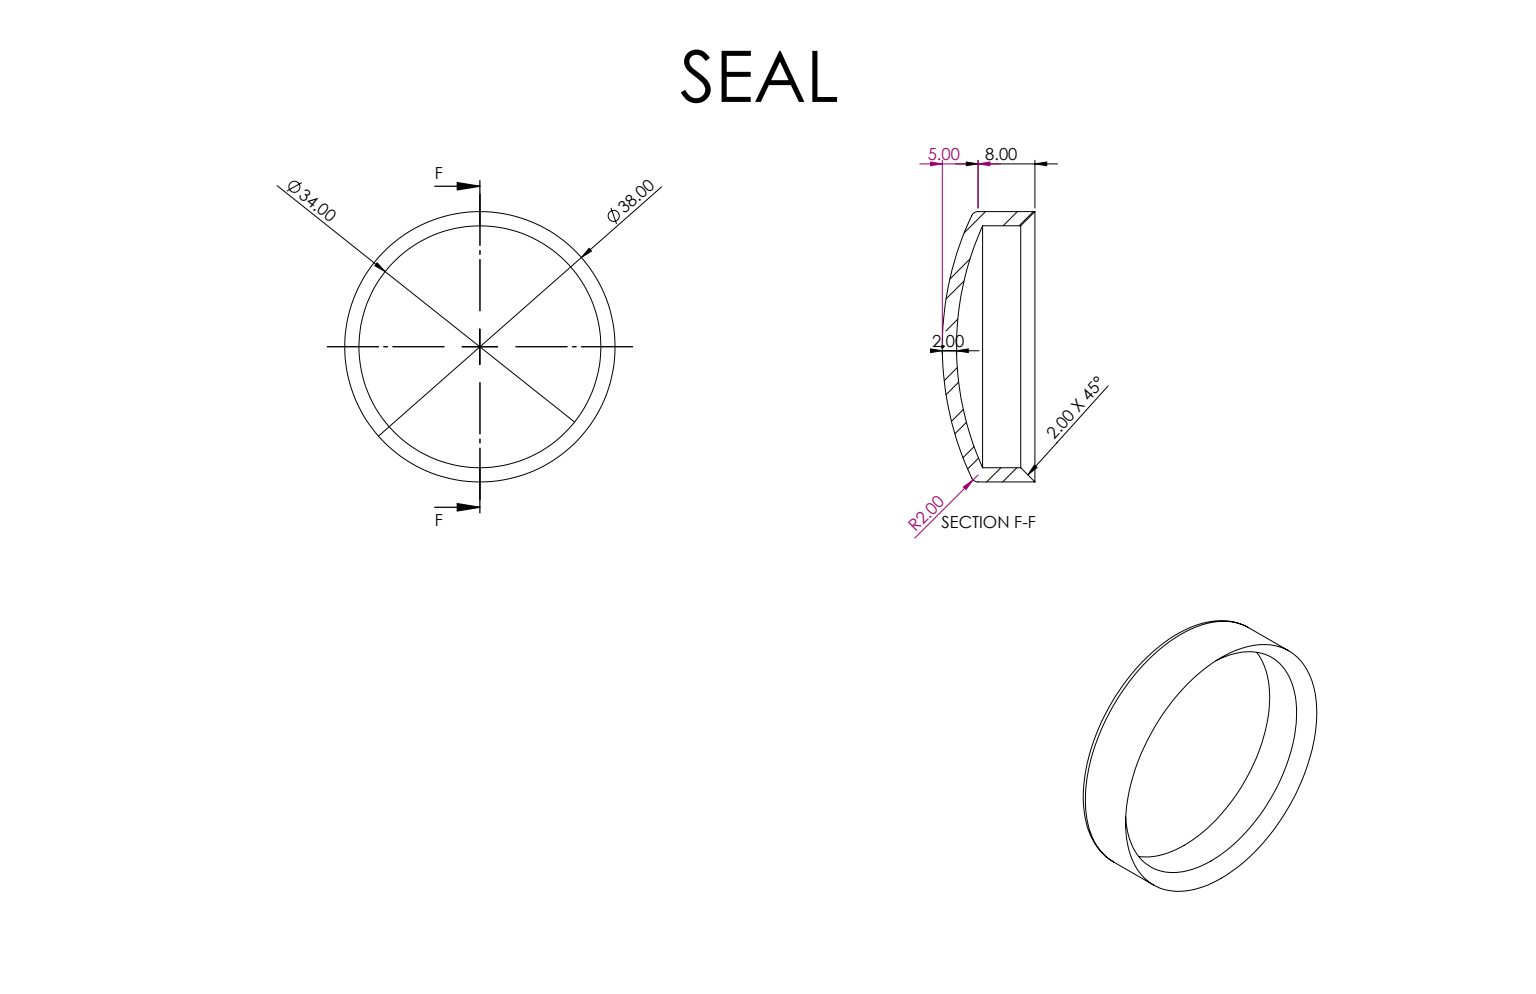
ISO-10303-21;
HEADER;
FILE_DESCRIPTION (('STEP AP214'),
    '1' );
FILE_NAME ('SEAL.step',
    '2026-10-24T00:51:42',
    ( '' ),
    ( '' ),
    'SwSTEP 2.0',
    'SolidWorks 2025',
    '' );
FILE_SCHEMA (( 'AUTOMOTIVE_DESIGN' ));
ENDSEC;

DATA;
#11=DIRECTION ( 'NONE',  ( -0.000000000000000000, 1.000000000000000000, -0.000000000000000000 ) ) ;
#27=ORIENTED_EDGE ( 'NONE', *, *, #9694, .T. ) ;
#55=ORIENTED_EDGE ( 'NONE', *, *, #16648, .F. ) ;
#84=APPLICATION_CONTEXT ( 'automotive_design' ) ;
#87=DIRECTION ( 'NONE',  ( -1.000000000000000000, 0.000000000000000000, 0.000000000000000000 ) ) ;
#107=CARTESIAN_POINT ( 'NONE',  ( 4.928914132345181612E-15, 5.025303850726727362, -19.00000000000000355 ) ) ;
#177=LINE ( 'NONE', #21385, #3523 ) ;
#207=DIRECTION ( 'NONE',  ( 1.000000000000000000, 0.000000000000000000, 1.224646799147352961E-16 ) ) ;
#305=AXIS2_PLACEMENT_3D ( 'NONE', #12969, #11033, #9203 ) ;
#323=CARTESIAN_POINT ( 'NONE',  ( 4.683984772515712893E-15, 6.000000000000019540, -17.00000000000000355 ) ) ;
#349=VERTEX_POINT ( 'NONE', #14379 ) ;
#459=CARTESIAN_POINT ( 'NONE',  ( 8.206546567640634603E-16, -5.025303850726727362, 0.000000000000000000 ) ) ;
#475=( NAMED_UNIT ( * ) SI_UNIT ( $, .STERADIAN. ) SOLID_ANGLE_UNIT ( ) );
#537=DIRECTION ( 'NONE',  ( -0.000000000000000000, 1.000000000000000000, -0.000000000000000000 ) ) ;
#567=CIRCLE ( 'NONE', #13356, 0.9999999999999974465 ) ;
#614=ORIENTED_EDGE ( 'NONE', *, *, #18115, .T. ) ;
#643=AXIS2_PLACEMENT_3D ( 'NONE', #1476, #22451, #1241 ) ;
#645=EDGE_CURVE ( 'NONE', #4303, #9582, #20624, .T. ) ;
#674=AXIS2_PLACEMENT_3D ( 'NONE', #11250, #20311, #16409 ) ;
#702=CIRCLE ( 'NONE', #18268, 41.25806096964026892 ) ;
#740=EDGE_CURVE ( 'NONE', #9582, #4006, #18031, .T. ) ;
#760=FACE_OUTER_BOUND ( 'NONE', #5319, .T. ) ;
#913=DIRECTION ( 'NONE',  ( 0.000000000000000000, 0.000000000000000000, 1.000000000000000000 ) ) ;
#941=DIRECTION ( 'NONE',  ( 0.000000000000000000, 0.000000000000000000, 1.000000000000000000 ) ) ;
#1145=ORIENTED_EDGE ( 'NONE', *, *, #20842, .T. ) ;
#1157=VERTEX_POINT ( 'NONE', #459 ) ;
#1241=DIRECTION ( 'NONE',  ( 0.000000000000000000, 0.000000000000000000, 1.000000000000000000 ) ) ;
#1412=AXIS2_PLACEMENT_3D ( 'NONE', #14691, #11146, #21698 ) ;
#1476=CARTESIAN_POINT ( 'NONE',  ( 2.602085213965210642E-15, 0.6398376396478597794, 0.000000000000000000 ) ) ;
#1503=AXIS2_PLACEMENT_3D ( 'NONE', #16634, #6320, #941 ) ;
#1549=FACE_OUTER_BOUND ( 'NONE', #14128, .T. ) ;
#1613=ORIENTED_EDGE ( 'NONE', *, *, #6289, .T. ) ;
#1626=DIRECTION ( 'NONE',  ( 0.000000000000000000, 0.000000000000000000, 1.000000000000000000 ) ) ;
#1631=VECTOR ( 'NONE', #2464, 1000.000000000000000 ) ;
#1646=CLOSED_SHELL ( 'NONE', ( #14748, #6755, #20935, #16987, #10183, #8647, #5905, #22314, #11559, #16889, #11992, #8653 ) ) ;
#1648=CARTESIAN_POINT ( 'NONE',  ( 0.000000000000000000, 0.000000000000000000, 0.000000000000000000 ) ) ;
#1670=DIRECTION ( 'NONE',  ( -0.000000000000000000, 1.000000000000000000, -0.000000000000000000 ) ) ;
#1672=ORIENTED_EDGE ( 'NONE', *, *, #19117, .T. ) ;
#1716=ORIENTED_EDGE ( 'NONE', *, *, #18989, .F. ) ;
#1776=CYLINDRICAL_SURFACE ( 'NONE', #3534, 17.00000000000000711 ) ;
#1824=CARTESIAN_POINT ( 'NONE',  ( 3.469446951953614189E-15, 38.23275711891355400, 0.000000000000000000 ) ) ;
#2001=CYLINDRICAL_SURFACE ( 'NONE', #17292, 17.00000000000000711 ) ;
#2006=ORIENTED_EDGE ( 'NONE', *, *, #3561, .T. ) ;
#2062=CARTESIAN_POINT ( 'NONE',  ( 4.683984772515712893E-15, 5.025303850726727362, -17.00000000000000711 ) ) ;
#2208=TOROIDAL_SURFACE ( 'NONE', #18687, 18.00000000000000711, 0.9999999999999985567 ) ;
#2352=DIRECTION ( 'NONE',  ( 0.000000000000000000, 0.000000000000000000, 1.000000000000000000 ) ) ;
#2365=EDGE_CURVE ( 'NONE', #18225, #21604, #22661, .T. ) ;
#2464=DIRECTION ( 'NONE',  ( 8.659560562354982162E-17, 0.7071067811865435759, -0.7071067811865515695 ) ) ;
#2537=ORIENTED_EDGE ( 'NONE', *, *, #19117, .F. ) ;
#2538=DIRECTION ( 'NONE',  ( -0.000000000000000000, 1.000000000000000000, -0.000000000000000000 ) ) ;
#2549=EDGE_LOOP ( 'NONE', ( #4013, #10589, #21393, #55, #10631 ) ) ;
#2553=UNCERTAINTY_MEASURE_WITH_UNIT (LENGTH_MEASURE( 1.000000000000000082E-05 ), #19676, 'distance_accuracy_value', 'NONE');
#2657=CARTESIAN_POINT ( 'NONE',  ( 3.469446951953614189E-15, 6.776263578034402713E-17, 18.00000000000000711 ) ) ;
#2946=ORIENTED_EDGE ( 'NONE', *, *, #645, .T. ) ;
#3114=ORIENTED_EDGE ( 'NONE', *, *, #17594, .T. ) ;
#3204=EDGE_LOOP ( 'NONE', ( #1613, #11629, #3342, #12290 ) ) ;
#3294=AXIS2_PLACEMENT_3D ( 'NONE', #17858, #14052, #207 ) ;
#3342=ORIENTED_EDGE ( 'NONE', *, *, #9694, .F. ) ;
#3523=VECTOR ( 'NONE', #21160, 1000.000000000000000 ) ;
#3534=AXIS2_PLACEMENT_3D ( 'NONE', #21241, #17677, #19191 ) ;
#3561=EDGE_CURVE ( 'NONE', #349, #8848, #15819, .T. ) ;
#3567=CARTESIAN_POINT ( 'NONE',  ( 2.602085213965210642E-15, -0.9047447100419790944, 0.000000000000000000 ) ) ;
#3577=ORIENTED_EDGE ( 'NONE', *, *, #8483, .F. ) ;
#3667=CARTESIAN_POINT ( 'NONE',  ( 2.602085213965210642E-15, 0.6398376396478597794, 0.000000000000000000 ) ) ;
#3686=DIRECTION ( 'NONE',  ( -0.000000000000000000, 1.000000000000000000, -0.000000000000000000 ) ) ;
#3801=LINE ( 'NONE', #15709, #15952 ) ;
#3881=CARTESIAN_POINT ( 'NONE',  ( 3.469446951953614189E-15, 6.776263578034402713E-17, 0.000000000000000000 ) ) ;
#3999=DIRECTION ( 'NONE',  ( 0.000000000000000000, 0.000000000000000000, 1.000000000000000000 ) ) ;
#4003=PRODUCT_DEFINITION_FORMATION_WITH_SPECIFIED_SOURCE ( 'ANY', '', #20116, .NOT_KNOWN. ) ;
#4006=VERTEX_POINT ( 'NONE', #12899 ) ;
#4013=ORIENTED_EDGE ( 'NONE', *, *, #18989, .T. ) ;
#4107=FACE_OUTER_BOUND ( 'NONE', #6243, .T. ) ;
#4126=ORIENTED_EDGE ( 'NONE', *, *, #7210, .F. ) ;
#4148=DIRECTION ( 'NONE',  ( 0.000000000000000000, 0.000000000000000000, 1.000000000000000000 ) ) ;
#4202=( NAMED_UNIT ( * ) PLANE_ANGLE_UNIT ( ) SI_UNIT ( $, .RADIAN. ) );
#4260=DIRECTION ( 'NONE',  ( -1.000000000000000000, 0.000000000000000000, 0.000000000000000000 ) ) ;
#4284=AXIS2_PLACEMENT_3D ( 'NONE', #11457, #2538, #6199 ) ;
#4303=VERTEX_POINT ( 'NONE', #19750 ) ;
#4521=CIRCLE ( 'NONE', #6705, 17.00000000000000711 ) ;
#4537=EDGE_CURVE ( 'NONE', #349, #4006, #12258, .T. ) ;
#4551=AXIS2_PLACEMENT_3D ( 'NONE', #5699, #537, #14507 ) ;
#4853=ORIENTED_EDGE ( 'NONE', *, *, #12898, .F. ) ;
#4904=ORIENTED_EDGE ( 'NONE', *, *, #18911, .F. ) ;
#5019=DIRECTION ( 'NONE',  ( -0.000000000000000000, -0.000000000000000000, -1.000000000000000000 ) ) ;
#5109=( GEOMETRIC_REPRESENTATION_CONTEXT ( 3 ) GLOBAL_UNCERTAINTY_ASSIGNED_CONTEXT ( ( #22046 ) ) GLOBAL_UNIT_ASSIGNED_CONTEXT ( ( #17664, #12495, #475 ) ) REPRESENTATION_CONTEXT ( 'NONE', 'WORKASPACE' ) );
#5149=ORIENTED_EDGE ( 'NONE', *, *, #3561, .F. ) ;
#5319=EDGE_LOOP ( 'NONE', ( #12095, #20816, #15192, #3114 ) ) ;
#5331=CARTESIAN_POINT ( 'NONE',  ( 2.602085213965210642E-15, 5.025303850726727362, 0.000000000000000000 ) ) ;
#5482=DIRECTION ( 'NONE',  ( -1.000000000000000000, 0.000000000000000000, 0.000000000000000000 ) ) ;
#5699=CARTESIAN_POINT ( 'NONE',  ( 2.602085213965210642E-15, 5.025303850726727362, 0.000000000000000000 ) ) ;
#5756=CIRCLE ( 'NONE', #643, 17.00000000000000711 ) ;
#5827=DIRECTION ( 'NONE',  ( 1.000000000000000000, 0.000000000000000000, 1.224646799147353207E-16 ) ) ;
#5852=ORIENTED_EDGE ( 'NONE', *, *, #2365, .F. ) ;
#5905=ADVANCED_FACE ( 'NONE', ( #4107 ), #17962, .T. ) ;
#5925=FACE_OUTER_BOUND ( 'NONE', #3204, .T. ) ;
#6086=APPLICATION_CONTEXT ( 'automotive_design' ) ;
#6106=VERTEX_POINT ( 'NONE', #9592 ) ;
#6199=DIRECTION ( 'NONE',  ( 0.000000000000000000, 0.000000000000000000, 1.000000000000000000 ) ) ;
#6243=EDGE_LOOP ( 'NONE', ( #16437, #8303, #5852, #1716 ) ) ;
#6261=EDGE_CURVE ( 'NONE', #15308, #12719, #8354, .T. ) ;
#6289=EDGE_CURVE ( 'NONE', #8848, #349, #20074, .T. ) ;
#6295=DIRECTION ( 'NONE',  ( 0.000000000000000000, 0.000000000000000000, 1.000000000000000000 ) ) ;
#6320=DIRECTION ( 'NONE',  ( -0.000000000000000000, 1.000000000000000000, -0.000000000000000000 ) ) ;
#6322=FACE_OUTER_BOUND ( 'NONE', #10656, .T. ) ;
#6380=DIRECTION ( 'NONE',  ( 0.000000000000000000, 0.000000000000000000, 1.000000000000000000 ) ) ;
#6500=DIRECTION ( 'NONE',  ( 0.000000000000000000, 0.000000000000000000, 1.000000000000000000 ) ) ;
#6616=CARTESIAN_POINT ( 'NONE',  ( 3.469446951953614189E-15, 38.23275711891355400, 0.000000000000000000 ) ) ;
#6679=CARTESIAN_POINT ( 'NONE',  ( 2.602085213965210642E-15, 7.999999999999994671, 0.000000000000000000 ) ) ;
#6695=DIRECTION ( 'NONE',  ( -0.000000000000000000, 1.000000000000000000, -0.000000000000000000 ) ) ;
#6705=AXIS2_PLACEMENT_3D ( 'NONE', #16325, #21606, #2352 ) ;
#6745=VERTEX_POINT ( 'NONE', #21629 ) ;
#6755=ADVANCED_FACE ( 'NONE', ( #5925 ), #13005, .T. ) ;
#6784=CARTESIAN_POINT ( 'NONE',  ( 3.469446951953614189E-15, 6.776263578034402713E-17, 0.000000000000000000 ) ) ;
#6913=ORIENTED_EDGE ( 'NONE', *, *, #740, .F. ) ;
#6934=CARTESIAN_POINT ( 'NONE',  ( 2.602085213965210642E-15, 0.000000000000000000, 19.00000000000000355 ) ) ;
#6992=CIRCLE ( 'NONE', #1503, 18.42595423422130452 ) ;
#7072=AXIS2_PLACEMENT_3D ( 'NONE', #21001, #8845, #8618 ) ;
#7079=FACE_OUTER_BOUND ( 'NONE', #8434, .T. ) ;
#7193=CARTESIAN_POINT ( 'NONE',  ( 3.469446951953614189E-15, 38.23275711891355400, 0.000000000000000000 ) ) ;
#7210=EDGE_CURVE ( 'NONE', #12719, #17759, #4521, .T. ) ;
#7233=DIRECTION ( 'NONE',  ( 0.000000000000000000, 0.7071067811865435759, 0.7071067811865515695 ) ) ;
#7237=VECTOR ( 'NONE', #3686, 1000.000000000000000 ) ;
#7290=MECHANICAL_DESIGN_GEOMETRIC_PRESENTATION_REPRESENTATION('',(#8749),#19010);
#7340=CARTESIAN_POINT ( 'NONE',  ( -17.00000000000000711, 0.6398376396478597794, 0.000000000000000000 ) ) ;
#7439=PRODUCT_DEFINITION ( 'UNKNOWN', '', #4003, #19672 ) ;
#7813=EDGE_CURVE ( 'NONE', #16292, #4303, #22402, .T. ) ;
#7875=AXIS2_PLACEMENT_3D ( 'NONE', #6784, #14080, #1626 ) ;
#7907=CARTESIAN_POINT ( 'NONE',  ( 2.602085213965210642E-15, 6.000000000000019540, 0.000000000000000000 ) ) ;
#7963=EDGE_LOOP ( 'NONE', ( #13873, #2006, #8237, #2537 ) ) ;
#8005=AXIS2_PLACEMENT_3D ( 'NONE', #3567, #17533, #14067 ) ;
#8073=EDGE_CURVE ( 'NONE', #6745, #6106, #6992, .T. ) ;
#8237=ORIENTED_EDGE ( 'NONE', *, *, #15184, .T. ) ;
#8246=ORIENTED_EDGE ( 'NONE', *, *, #12898, .T. ) ;
#8303=ORIENTED_EDGE ( 'NONE', *, *, #18398, .T. ) ;
#8354=CIRCLE ( 'NONE', #1412, 41.25806096964028313 ) ;
#8434=EDGE_LOOP ( 'NONE', ( #18614, #9584, #8246, #18274, #5149 ) ) ;
#8483=EDGE_CURVE ( 'NONE', #9582, #4303, #20499, .T. ) ;
#8490=ORIENTED_EDGE ( 'NONE', *, *, #645, .F. ) ;
#8618=DIRECTION ( 'NONE',  ( 0.000000000000000000, 0.000000000000000000, 1.000000000000000000 ) ) ;
#8632=CARTESIAN_POINT ( 'NONE',  ( 2.602085213965210642E-15, 5.025303850726727362, 17.00000000000000711 ) ) ;
#8647=ADVANCED_FACE ( 'NONE', ( #21290 ), #12559, .T. ) ;
#8653=ADVANCED_FACE ( 'NONE', ( #7079 ), #2208, .T. ) ;
#8672=CONICAL_SURFACE ( 'NONE', #4284, 17.00000000000000355, 0.7853981633974539411 ) ;
#8749=STYLED_ITEM('',(#22741),#17806);
#8773=CARTESIAN_POINT ( 'NONE',  ( 2.602085213965210642E-15, 6.000000000000019540, 0.000000000000000000 ) ) ;
#8845=DIRECTION ( 'NONE',  ( -0.000000000000000000, 1.000000000000000000, -0.000000000000000000 ) ) ;
#8848=VERTEX_POINT ( 'NONE', #6934 ) ;
#8885=AXIS2_PLACEMENT_3D ( 'NONE', #21552, #21895, #913 ) ;
#9030=CARTESIAN_POINT ( 'NONE',  ( 5.673811190418850800E-15, 6.776263578034402713E-17, -18.00000000000000711 ) ) ;
#9048=AXIS2_PLACEMENT_3D ( 'NONE', #12261, #11, #19152 ) ;
#9203=DIRECTION ( 'NONE',  ( 0.000000000000000000, 0.000000000000000000, 1.000000000000000000 ) ) ;
#9422=VERTEX_POINT ( 'NONE', #7340 ) ;
#9560=ORIENTED_EDGE ( 'NONE', *, *, #6261, .F. ) ;
#9575=DIRECTION ( 'NONE',  ( 0.000000000000000000, 0.000000000000000000, 1.000000000000000000 ) ) ;
#9582=VERTEX_POINT ( 'NONE', #323 ) ;
#9584=ORIENTED_EDGE ( 'NONE', *, *, #2365, .T. ) ;
#9592=CARTESIAN_POINT ( 'NONE',  ( 18.42595423422130452, -0.9047447100419843125, 2.256528587417473578E-15 ) ) ;
#9599=CARTESIAN_POINT ( 'NONE',  ( 5.761125704852336857E-15, -0.9047447100419790944, -18.42595423422130452 ) ) ;
#9675=EDGE_LOOP ( 'NONE', ( #3577, #13696, #1672, #14952 ) ) ;
#9694=EDGE_CURVE ( 'NONE', #21260, #4006, #22251, .T. ) ;
#9823=FACE_OUTER_BOUND ( 'NONE', #17736, .T. ) ;
#9992=CARTESIAN_POINT ( 'NONE',  ( 2.602085213965210642E-15, 0.6398376396478597794, 17.00000000000000711 ) ) ;
#10140=AXIS2_PLACEMENT_3D ( 'NONE', #15413, #13811, #6500 ) ;
#10183=ADVANCED_FACE ( 'NONE', ( #760 ), #12993, .F. ) ;
#10222=CIRCLE ( 'NONE', #3294, 43.25806096964028313 ) ;
#10247=AXIS2_PLACEMENT_3D ( 'NONE', #1824, #19359, #87 ) ;
#10280=CARTESIAN_POINT ( 'NONE',  ( -18.42595423422129741, -0.9047447100419843125, 0.000000000000000000 ) ) ;
#10287=DIRECTION ( 'NONE',  ( -0.000000000000000000, 1.000000000000000000, -0.000000000000000000 ) ) ;
#10589=ORIENTED_EDGE ( 'NONE', *, *, #17660, .T. ) ;
#10631=ORIENTED_EDGE ( 'NONE', *, *, #8073, .T. ) ;
#10656=EDGE_LOOP ( 'NONE', ( #9560, #14306, #19115, #11443 ) ) ;
#10907=SHAPE_REPRESENTATION ( 'SEAL', ( #18273 ), #5109 ) ;
#10952=( NAMED_UNIT ( * ) SI_UNIT ( $, .STERADIAN. ) SOLID_ANGLE_UNIT ( ) );
#11033=DIRECTION ( 'NONE',  ( -0.000000000000000000, 1.000000000000000000, -0.000000000000000000 ) ) ;
#11146=DIRECTION ( 'NONE',  ( -1.224646799147353207E-16, 0.000000000000000000, 1.000000000000000000 ) ) ;
#11250=CARTESIAN_POINT ( 'NONE',  ( 3.469446951953614189E-15, 38.23275711891355400, 0.000000000000000000 ) ) ;
#11268=AXIS2_PLACEMENT_3D ( 'NONE', #20010, #9575, #13444 ) ;
#11322=CARTESIAN_POINT ( 'NONE',  ( 2.602085213965210642E-15, 7.999999999999994671, 19.00000000000000355 ) ) ;
#11339=ORIENTED_EDGE ( 'NONE', *, *, #22505, .F. ) ;
#11443=ORIENTED_EDGE ( 'NONE', *, *, #21508, .T. ) ;
#11457=CARTESIAN_POINT ( 'NONE',  ( 2.602085213965210642E-15, 6.000000000000019540, 0.000000000000000000 ) ) ;
#11559=ADVANCED_FACE ( 'NONE', ( #1549 ), #2001, .F. ) ;
#11629=ORIENTED_EDGE ( 'NONE', *, *, #4537, .T. ) ;
#11899=CIRCLE ( 'NONE', #17756, 0.9999999999999974465 ) ;
#11947=CYLINDRICAL_SURFACE ( 'NONE', #7072, 19.00000000000000355 ) ;
#11992=ADVANCED_FACE ( 'NONE', ( #15817 ), #11947, .T. ) ;
#12095=ORIENTED_EDGE ( 'NONE', *, *, #17750, .F. ) ;
#12146=PRODUCT_CONTEXT ( 'NONE', #84, 'mechanical' ) ;
#12151=LINE ( 'NONE', #2062, #7237 ) ;
#12152=CARTESIAN_POINT ( 'NONE',  ( 2.602085213965210642E-15, 0.6398376396478597794, 0.000000000000000000 ) ) ;
#12258=LINE ( 'NONE', #107, #20185 ) ;
#12261=CARTESIAN_POINT ( 'NONE',  ( 2.602085213965210642E-15, -0.9047447100419790944, 0.000000000000000000 ) ) ;
#12290=ORIENTED_EDGE ( 'NONE', *, *, #15184, .F. ) ;
#12462=CARTESIAN_POINT ( 'NONE',  ( 17.00000000000001421, 0.6398376396478597794, 2.081899558550501463E-15 ) ) ;
#12495=( NAMED_UNIT ( * ) PLANE_ANGLE_UNIT ( ) SI_UNIT ( $, .RADIAN. ) );
#12507=FACE_OUTER_BOUND ( 'NONE', #22174, .T. ) ;
#12559=SPHERICAL_SURFACE ( 'NONE', #10247, 43.25806096964027603 ) ;
#12719=VERTEX_POINT ( 'NONE', #12462 ) ;
#12898=EDGE_CURVE ( 'NONE', #21604, #6745, #13736, .T. ) ;
#12899=CARTESIAN_POINT ( 'NONE',  ( 4.928914132345180823E-15, 7.999999999999994671, -19.00000000000000355 ) ) ;
#12969=CARTESIAN_POINT ( 'NONE',  ( 2.602085213965210642E-15, 0.000000000000000000, 0.000000000000000000 ) ) ;
#12993=SPHERICAL_SURFACE ( 'NONE', #11268, 41.25806096964027603 ) ;
#13005=CYLINDRICAL_SURFACE ( 'NONE', #4551, 19.00000000000000355 ) ;
#13154=ADVANCED_BREP_SHAPE_REPRESENTATION ( '', ( #17806, #18273 ), #5109 ) ;
#13231=CARTESIAN_POINT ( 'NONE',  ( 2.602085213965210642E-15, 6.000000000000019540, 0.000000000000000000 ) ) ;
#13356=AXIS2_PLACEMENT_3D ( 'NONE', #2657, #4260, #4148 ) ;
#13369=ORIENTED_EDGE ( 'NONE', *, *, #8483, .T. ) ;
#13444=DIRECTION ( 'NONE',  ( -1.000000000000000000, 0.000000000000000000, 0.000000000000000000 ) ) ;
#13474=CIRCLE ( 'NONE', #18985, 17.00000000000000711 ) ;
#13578=DIRECTION ( 'NONE',  ( -0.000000000000000000, -0.000000000000000000, -1.000000000000000000 ) ) ;
#13654=AXIS2_PLACEMENT_3D ( 'NONE', #8773, #1670, #15628 ) ;
#13696=ORIENTED_EDGE ( 'NONE', *, *, #740, .T. ) ;
#13736=CIRCLE ( 'NONE', #16690, 18.42595423422130452 ) ;
#13811=DIRECTION ( 'NONE',  ( -0.000000000000000000, 1.000000000000000000, -0.000000000000000000 ) ) ;
#13873=ORIENTED_EDGE ( 'NONE', *, *, #4537, .F. ) ;
#13924=DIRECTION ( 'NONE',  ( -1.000000000000000000, 0.000000000000000000, 0.000000000000000000 ) ) ;
#14052=DIRECTION ( 'NONE',  ( -1.224646799147353207E-16, 0.000000000000000000, 1.000000000000000000 ) ) ;
#14067=DIRECTION ( 'NONE',  ( 0.000000000000000000, 0.000000000000000000, 1.000000000000000000 ) ) ;
#14069=AXIS2_PLACEMENT_3D ( 'NONE', #3667, #10287, #20963 ) ;
#14080=DIRECTION ( 'NONE',  ( -0.000000000000000000, 1.000000000000000000, -0.000000000000000000 ) ) ;
#14128=EDGE_LOOP ( 'NONE', ( #4904, #4126, #22022, #16169, #2946 ) ) ;
#14306=ORIENTED_EDGE ( 'NONE', *, *, #17750, .T. ) ;
#14379=CARTESIAN_POINT ( 'NONE',  ( 4.928914132345181612E-15, 0.000000000000000000, -19.00000000000000355 ) ) ;
#14507=DIRECTION ( 'NONE',  ( 0.000000000000000000, 0.000000000000000000, 1.000000000000000000 ) ) ;
#14592=CARTESIAN_POINT ( 'NONE',  ( 4.683984772515711316E-15, 6.000000000000019540, -17.00000000000000355 ) ) ;
#14618=CIRCLE ( 'NONE', #22336, 43.25806096964026892 ) ;
#14689=EDGE_LOOP ( 'NONE', ( #20559, #614, #22461, #4853 ) ) ;
#14691=CARTESIAN_POINT ( 'NONE',  ( 3.469446951953614189E-15, 38.23275711891355400, 0.000000000000000000 ) ) ;
#14748=ADVANCED_FACE ( 'NONE', ( #21524 ), #19949, .T. ) ;
#14859=CARTESIAN_POINT ( 'NONE',  ( 2.602085213965210642E-15, -0.9047447100419790944, 0.000000000000000000 ) ) ;
#14952=ORIENTED_EDGE ( 'NONE', *, *, #20842, .F. ) ;
#14973=DIRECTION ( 'NONE',  ( 0.000000000000000000, 0.000000000000000000, 1.000000000000000000 ) ) ;
#15009=VECTOR ( 'NONE', #6695, 1000.000000000000000 ) ;
#15184=EDGE_CURVE ( 'NONE', #8848, #21260, #177, .T. ) ;
#15192=ORIENTED_EDGE ( 'NONE', *, *, #7210, .T. ) ;
#15308=VERTEX_POINT ( 'NONE', #18173 ) ;
#15413=CARTESIAN_POINT ( 'NONE',  ( 2.602085213965210642E-15, 7.999999999999994671, 0.000000000000000000 ) ) ;
#15454=SHAPE_DEFINITION_REPRESENTATION ( #21955, #10907 ) ;
#15491=DIRECTION ( 'NONE',  ( 0.000000000000000000, 0.000000000000000000, 1.000000000000000000 ) ) ;
#15628=DIRECTION ( 'NONE',  ( 0.000000000000000000, 0.000000000000000000, 1.000000000000000000 ) ) ;
#15631=AXIS2_PLACEMENT_3D ( 'NONE', #6679, #22618, #20654 ) ;
#15709=CARTESIAN_POINT ( 'NONE',  ( 2.602085213965210642E-15, 6.000000000000019540, 17.00000000000000355 ) ) ;
#15777=DIRECTION ( 'NONE',  ( -0.000000000000000000, 1.000000000000000000, -0.000000000000000000 ) ) ;
#15817=FACE_OUTER_BOUND ( 'NONE', #7963, .T. ) ;
#15819=CIRCLE ( 'NONE', #8885, 19.00000000000000355 ) ;
#15949=AXIS2_PLACEMENT_3D ( 'NONE', #13231, #22089, #6380 ) ;
#15952=VECTOR ( 'NONE', #7233, 1000.000000000000000 ) ;
#16169=ORIENTED_EDGE ( 'NONE', *, *, #7813, .T. ) ;
#16292=VERTEX_POINT ( 'NONE', #9992 ) ;
#16325=CARTESIAN_POINT ( 'NONE',  ( 2.602085213965210642E-15, 0.6398376396478597794, 0.000000000000000000 ) ) ;
#16409=DIRECTION ( 'NONE',  ( -1.000000000000000000, 0.000000000000000000, 0.000000000000000000 ) ) ;
#16437=ORIENTED_EDGE ( 'NONE', *, *, #18115, .F. ) ;
#16634=CARTESIAN_POINT ( 'NONE',  ( 2.602085213965210642E-15, -0.9047447100419790944, 0.000000000000000000 ) ) ;
#16648=EDGE_CURVE ( 'NONE', #6745, #8848, #567, .T. ) ;
#16690=AXIS2_PLACEMENT_3D ( 'NONE', #14859, #16831, #14973 ) ;
#16831=DIRECTION ( 'NONE',  ( -0.000000000000000000, 1.000000000000000000, -0.000000000000000000 ) ) ;
#16889=ADVANCED_FACE ( 'NONE', ( #9823 ), #18514, .F. ) ;
#16987=ADVANCED_FACE ( 'NONE', ( #12507 ), #1776, .F. ) ;
#16993=DIRECTION ( 'NONE',  ( 1.000000000000000000, 0.000000000000000000, 0.000000000000000000 ) ) ;
#17193=DIRECTION ( 'NONE',  ( -0.000000000000000000, 1.000000000000000000, -0.000000000000000000 ) ) ;
#17292=AXIS2_PLACEMENT_3D ( 'NONE', #5331, #21141, #17689 ) ;
#17533=DIRECTION ( 'NONE',  ( -0.000000000000000000, 1.000000000000000000, -0.000000000000000000 ) ) ;
#17535=DIRECTION ( 'NONE',  ( -0.000000000000000000, 1.000000000000000000, -0.000000000000000000 ) ) ;
#17584=AXIS2_PLACEMENT_3D ( 'NONE', #7907, #22002, #6295 ) ;
#17594=EDGE_CURVE ( 'NONE', #17759, #9422, #19230, .T. ) ;
#17641=DIRECTION ( 'NONE',  ( 0.000000000000000000, 0.000000000000000000, 1.000000000000000000 ) ) ;
#17660=EDGE_CURVE ( 'NONE', #18225, #349, #11899, .T. ) ;
#17664=( LENGTH_UNIT ( ) NAMED_UNIT ( * ) SI_UNIT ( .MILLI., .METRE. ) );
#17677=DIRECTION ( 'NONE',  ( -0.000000000000000000, 1.000000000000000000, -0.000000000000000000 ) ) ;
#17689=DIRECTION ( 'NONE',  ( 0.000000000000000000, 0.000000000000000000, 1.000000000000000000 ) ) ;
#17733=DIRECTION ( 'NONE',  ( 0.000000000000000000, 0.000000000000000000, 1.000000000000000000 ) ) ;
#17736=EDGE_LOOP ( 'NONE', ( #6913, #8490, #1145, #27 ) ) ;
#17750=EDGE_CURVE ( 'NONE', #15308, #9422, #702, .T. ) ;
#17756=AXIS2_PLACEMENT_3D ( 'NONE', #9030, #5827, #18070 ) ;
#17759=VERTEX_POINT ( 'NONE', #19450 ) ;
#17806=MANIFOLD_SOLID_BREP ( 'Revolve1', #1646 ) ;
#17858=CARTESIAN_POINT ( 'NONE',  ( 3.469446951953614189E-15, 38.23275711891355400, 0.000000000000000000 ) ) ;
#17962=SPHERICAL_SURFACE ( 'NONE', #20444, 43.25806096964027603 ) ;
#18031=LINE ( 'NONE', #14592, #1631 ) ;
#18070=DIRECTION ( 'NONE',  ( 1.224646799147353700E-16, 0.000000000000000000, -1.000000000000000000 ) ) ;
#18115=EDGE_CURVE ( 'NONE', #1157, #6106, #10222, .T. ) ;
#18173=CARTESIAN_POINT ( 'NONE',  ( 9.431193366787989042E-16, -3.025303850726725141, 0.000000000000000000 ) ) ;
#18225=VERTEX_POINT ( 'NONE', #9599 ) ;
#18268=AXIS2_PLACEMENT_3D ( 'NONE', #22553, #5019, #13924 ) ;
#18273=AXIS2_PLACEMENT_3D ( 'NONE', #1648, #15491, #16993 ) ;
#18274=ORIENTED_EDGE ( 'NONE', *, *, #16648, .T. ) ;
#18398=EDGE_CURVE ( 'NONE', #1157, #21604, #14618, .T. ) ;
#18514=CONICAL_SURFACE ( 'NONE', #15949, 17.00000000000000355, 0.7853981633974539411 ) ;
#18614=ORIENTED_EDGE ( 'NONE', *, *, #17660, .F. ) ;
#18687=AXIS2_PLACEMENT_3D ( 'NONE', #3881, #15777, #3999 ) ;
#18911=EDGE_CURVE ( 'NONE', #17759, #9582, #12151, .T. ) ;
#18985=AXIS2_PLACEMENT_3D ( 'NONE', #12152, #17193, #17641 ) ;
#18989=EDGE_CURVE ( 'NONE', #6106, #18225, #20051, .T. ) ;
#19010=( GEOMETRIC_REPRESENTATION_CONTEXT ( 3 ) GLOBAL_UNCERTAINTY_ASSIGNED_CONTEXT ( ( #2553 ) ) GLOBAL_UNIT_ASSIGNED_CONTEXT ( ( #19676, #4202, #10952 ) ) REPRESENTATION_CONTEXT ( 'NONE', 'WORKASPACE' ) );
#19115=ORIENTED_EDGE ( 'NONE', *, *, #22505, .T. ) ;
#19117=EDGE_CURVE ( 'NONE', #4006, #21260, #22247, .T. ) ;
#19152=DIRECTION ( 'NONE',  ( 0.000000000000000000, 0.000000000000000000, 1.000000000000000000 ) ) ;
#19191=DIRECTION ( 'NONE',  ( 0.000000000000000000, 0.000000000000000000, 1.000000000000000000 ) ) ;
#19230=CIRCLE ( 'NONE', #14069, 17.00000000000000711 ) ;
#19359=DIRECTION ( 'NONE',  ( 0.000000000000000000, 0.000000000000000000, 1.000000000000000000 ) ) ;
#19450=CARTESIAN_POINT ( 'NONE',  ( 4.683984772515712893E-15, 0.6398376396478597794, -17.00000000000000711 ) ) ;
#19672=PRODUCT_DEFINITION_CONTEXT ( 'detailed design', #6086, 'design' ) ;
#19676=( LENGTH_UNIT ( ) NAMED_UNIT ( * ) SI_UNIT ( .MILLI., .METRE. ) );
#19750=CARTESIAN_POINT ( 'NONE',  ( 2.602085213965210642E-15, 6.000000000000019540, 17.00000000000000355 ) ) ;
#19949=TOROIDAL_SURFACE ( 'NONE', #7875, 18.00000000000000711, 0.9999999999999985567 ) ;
#20010=CARTESIAN_POINT ( 'NONE',  ( 3.469446951953614189E-15, 38.23275711891355400, 0.000000000000000000 ) ) ;
#20051=CIRCLE ( 'NONE', #9048, 18.42595423422130452 ) ;
#20074=CIRCLE ( 'NONE', #305, 19.00000000000000355 ) ;
#20080=SHAPE_REPRESENTATION_RELATIONSHIP ( 'NONE' , 'NONE' ,  #10907, #13154 ) ;
#20086=SPHERICAL_SURFACE ( 'NONE', #674, 41.25806096964027603 ) ;
#20116=PRODUCT ( 'SEAL', 'SEAL', '', ( #12146 ) ) ;
#20185=VECTOR ( 'NONE', #17535, 1000.000000000000000 ) ;
#20311=DIRECTION ( 'NONE',  ( 0.000000000000000000, 0.000000000000000000, 1.000000000000000000 ) ) ;
#20444=AXIS2_PLACEMENT_3D ( 'NONE', #7193, #17733, #5482 ) ;
#20499=CIRCLE ( 'NONE', #17584, 17.00000000000000355 ) ;
#20559=ORIENTED_EDGE ( 'NONE', *, *, #18398, .F. ) ;
#20593=DIRECTION ( 'NONE',  ( -1.000000000000000000, 0.000000000000000000, 0.000000000000000000 ) ) ;
#20624=CIRCLE ( 'NONE', #13654, 17.00000000000000355 ) ;
#20654=DIRECTION ( 'NONE',  ( 0.000000000000000000, 0.000000000000000000, 1.000000000000000000 ) ) ;
#20816=ORIENTED_EDGE ( 'NONE', *, *, #6261, .T. ) ;
#20842=EDGE_CURVE ( 'NONE', #4303, #21260, #3801, .T. ) ;
#20935=ADVANCED_FACE ( 'NONE', ( #21903 ), #8672, .F. ) ;
#20963=DIRECTION ( 'NONE',  ( 0.000000000000000000, 0.000000000000000000, 1.000000000000000000 ) ) ;
#21001=CARTESIAN_POINT ( 'NONE',  ( 2.602085213965210642E-15, 5.025303850726727362, 0.000000000000000000 ) ) ;
#21141=DIRECTION ( 'NONE',  ( -0.000000000000000000, 1.000000000000000000, -0.000000000000000000 ) ) ;
#21160=DIRECTION ( 'NONE',  ( -0.000000000000000000, 1.000000000000000000, -0.000000000000000000 ) ) ;
#21241=CARTESIAN_POINT ( 'NONE',  ( 2.602085213965210642E-15, 5.025303850726727362, 0.000000000000000000 ) ) ;
#21260=VERTEX_POINT ( 'NONE', #11322 ) ;
#21290=FACE_OUTER_BOUND ( 'NONE', #14689, .T. ) ;
#21385=CARTESIAN_POINT ( 'NONE',  ( 2.602085213965210642E-15, 5.025303850726727362, 19.00000000000000355 ) ) ;
#21393=ORIENTED_EDGE ( 'NONE', *, *, #6289, .F. ) ;
#21508=EDGE_CURVE ( 'NONE', #16292, #12719, #5756, .T. ) ;
#21524=FACE_OUTER_BOUND ( 'NONE', #2549, .T. ) ;
#21552=CARTESIAN_POINT ( 'NONE',  ( 2.602085213965210642E-15, 0.000000000000000000, 0.000000000000000000 ) ) ;
#21604=VERTEX_POINT ( 'NONE', #10280 ) ;
#21606=DIRECTION ( 'NONE',  ( -0.000000000000000000, 1.000000000000000000, -0.000000000000000000 ) ) ;
#21629=CARTESIAN_POINT ( 'NONE',  ( 3.469446951953614189E-15, -0.9047447100419790944, 18.42595423422130452 ) ) ;
#21650=ORIENTED_EDGE ( 'NONE', *, *, #18911, .T. ) ;
#21698=DIRECTION ( 'NONE',  ( 1.000000000000000000, 0.000000000000000000, 1.224646799147352961E-16 ) ) ;
#21761=ORIENTED_EDGE ( 'NONE', *, *, #7813, .F. ) ;
#21895=DIRECTION ( 'NONE',  ( -0.000000000000000000, 1.000000000000000000, -0.000000000000000000 ) ) ;
#21903=FACE_OUTER_BOUND ( 'NONE', #9675, .T. ) ;
#21955=PRODUCT_DEFINITION_SHAPE ( 'NONE', 'NONE',  #7439 ) ;
#22002=DIRECTION ( 'NONE',  ( -0.000000000000000000, 1.000000000000000000, -0.000000000000000000 ) ) ;
#22022=ORIENTED_EDGE ( 'NONE', *, *, #21508, .F. ) ;
#22046=UNCERTAINTY_MEASURE_WITH_UNIT (LENGTH_MEASURE( 1.000000000000000082E-05 ), #17664, 'distance_accuracy_value', 'NONE');
#22089=DIRECTION ( 'NONE',  ( -0.000000000000000000, 1.000000000000000000, -0.000000000000000000 ) ) ;
#22174=EDGE_LOOP ( 'NONE', ( #22340, #21650, #13369, #21761, #11339 ) ) ;
#22247=CIRCLE ( 'NONE', #15631, 19.00000000000000355 ) ;
#22251=CIRCLE ( 'NONE', #10140, 19.00000000000000355 ) ;
#22314=ADVANCED_FACE ( 'NONE', ( #6322 ), #20086, .F. ) ;
#22336=AXIS2_PLACEMENT_3D ( 'NONE', #6616, #13578, #20593 ) ;
#22340=ORIENTED_EDGE ( 'NONE', *, *, #17594, .F. ) ;
#22402=LINE ( 'NONE', #8632, #15009 ) ;
#22451=DIRECTION ( 'NONE',  ( -0.000000000000000000, 1.000000000000000000, -0.000000000000000000 ) ) ;
#22461=ORIENTED_EDGE ( 'NONE', *, *, #8073, .F. ) ;
#22505=EDGE_CURVE ( 'NONE', #9422, #16292, #13474, .T. ) ;
#22553=CARTESIAN_POINT ( 'NONE',  ( 3.469446951953614189E-15, 38.23275711891355400, 0.000000000000000000 ) ) ;
#22618=DIRECTION ( 'NONE',  ( -0.000000000000000000, 1.000000000000000000, -0.000000000000000000 ) ) ;
#22661=CIRCLE ( 'NONE', #8005, 18.42595423422130452 ) ;
#22735=COLOUR_RGB('Black',0.12,0.14,0.17);
#22736=FILL_AREA_STYLE_COLOUR('',#22735);
#22737=FILL_AREA_STYLE('',(#22736));
#22738=SURFACE_STYLE_FILL_AREA(#22737);
#22739=SURFACE_SIDE_STYLE('',(#22738));
#22740=SURFACE_STYLE_USAGE(.BOTH.,#22739);
#22741=PRESENTATION_STYLE_ASSIGNMENT((#22740));
ENDSEC;
END-ISO-10303-21;
